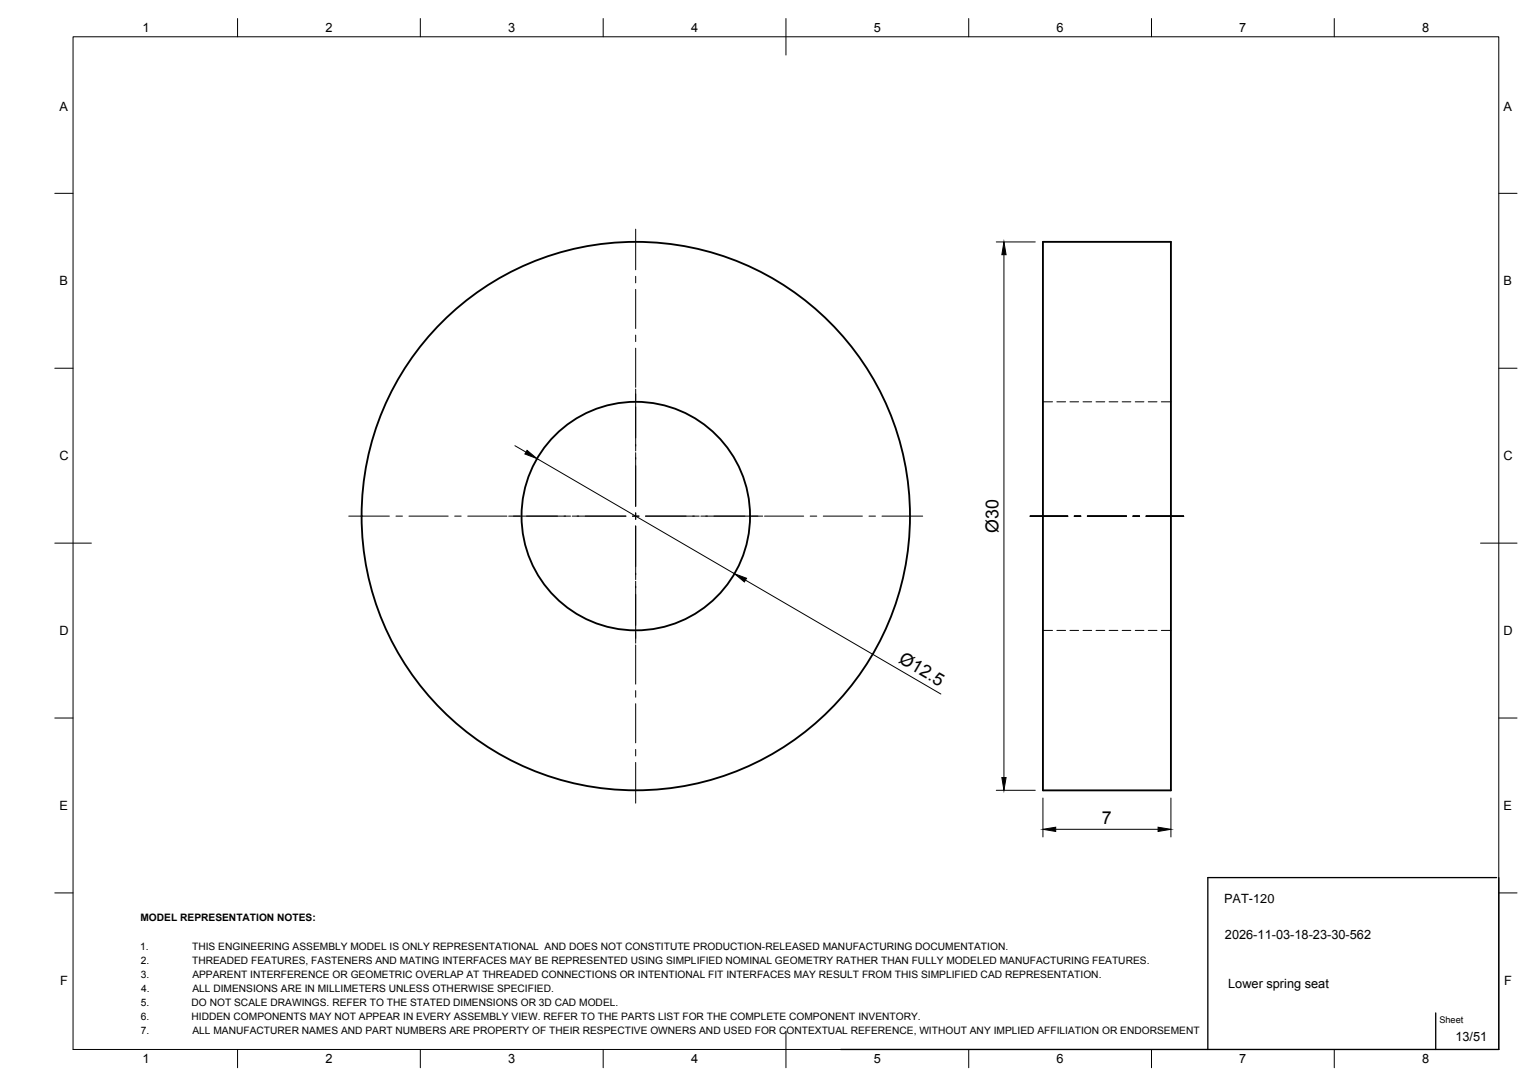
ISO-10303-21;
HEADER;
/* Generated by software containing ST-Developer
 * from STEP Tools, Inc. (www.steptools.com) 
 */

FILE_DESCRIPTION(
/* description */ ('Vibration shaker table dummy'),
/* implementation_level */ '2;1');

FILE_NAME(
/* name */ 'Lower spring seat.step',
/* time_stamp */ '2026-10-27T10:55:14-07:00',
/* author */ (''),
/* organization */ (''),
/* preprocessor_version */ 'ST-DEVELOPER v20.2',
/* originating_system */ 'Autodesk Translation Framework v15.17.0.0',
/* authorisation */ '');

FILE_SCHEMA (('AUTOMOTIVE_DESIGN { 1 0 10303 214 3 1 1 }'));
ENDSEC;

DATA;
#10=MECHANICAL_DESIGN_GEOMETRIC_PRESENTATION_REPRESENTATION('',(#694),#22394);
#602=SHAPE_REPRESENTATION_RELATIONSHIP('SRR','None',#22648,#648);
#648=ADVANCED_BREP_SHAPE_REPRESENTATION('',(#740),#22354);
#694=STYLED_ITEM('',(#22961),#740);
#740=MANIFOLD_SOLID_BREP('Body1',#9212);
#875=FACE_BOUND('',#2060,.T.);
#876=FACE_BOUND('',#2062,.T.);
#1122=PLANE('',#10011);
#1123=PLANE('',#10012);
#1459=FACE_OUTER_BOUND('',#2057,.T.);
#1460=FACE_OUTER_BOUND('',#2058,.T.);
#1461=FACE_OUTER_BOUND('',#2059,.T.);
#1462=FACE_OUTER_BOUND('',#2061,.T.);
#2057=EDGE_LOOP('',(#6810,#6811,#6812,#6813));
#2058=EDGE_LOOP('',(#6814,#6815,#6816,#6817));
#2059=EDGE_LOOP('',(#6818));
#2060=EDGE_LOOP('',(#6819));
#2061=EDGE_LOOP('',(#6820));
#2062=EDGE_LOOP('',(#6821));
#2788=LINE('',#14552,#3407);
#2789=LINE('',#14558,#3408);
#3407=VECTOR('',#11610,0.625);
#3408=VECTOR('',#11617,1.5);
#3976=CIRCLE('',#10006,0.625);
#3977=CIRCLE('',#10007,0.625);
#3978=CIRCLE('',#10009,1.5);
#3979=CIRCLE('',#10010,1.5);
#4555=VERTEX_POINT('',#14549);
#4556=VERTEX_POINT('',#14551);
#4557=VERTEX_POINT('',#14555);
#4558=VERTEX_POINT('',#14557);
#5398=EDGE_CURVE('',#4555,#4555,#3976,.T.);
#5399=EDGE_CURVE('',#4555,#4556,#2788,.T.);
#5400=EDGE_CURVE('',#4556,#4556,#3977,.T.);
#5401=EDGE_CURVE('',#4557,#4557,#3978,.T.);
#5402=EDGE_CURVE('',#4557,#4558,#2789,.T.);
#5403=EDGE_CURVE('',#4558,#4558,#3979,.T.);
#6810=ORIENTED_EDGE('',*,*,#5398,.F.);
#6811=ORIENTED_EDGE('',*,*,#5399,.T.);
#6812=ORIENTED_EDGE('',*,*,#5400,.T.);
#6813=ORIENTED_EDGE('',*,*,#5399,.F.);
#6814=ORIENTED_EDGE('',*,*,#5401,.F.);
#6815=ORIENTED_EDGE('',*,*,#5402,.T.);
#6816=ORIENTED_EDGE('',*,*,#5403,.T.);
#6817=ORIENTED_EDGE('',*,*,#5402,.F.);
#6818=ORIENTED_EDGE('',*,*,#5401,.T.);
#6819=ORIENTED_EDGE('',*,*,#5398,.T.);
#6820=ORIENTED_EDGE('',*,*,#5403,.F.);
#6821=ORIENTED_EDGE('',*,*,#5400,.F.);
#8562=CYLINDRICAL_SURFACE('',#10005,0.625);
#8563=CYLINDRICAL_SURFACE('',#10008,1.5);
#8824=ADVANCED_FACE('',(#1459),#8562,.F.);
#8825=ADVANCED_FACE('',(#1460),#8563,.T.);
#8826=ADVANCED_FACE('',(#1461,#875),#1122,.T.);
#8827=ADVANCED_FACE('',(#1462,#876),#1123,.F.);
#9212=CLOSED_SHELL('',(#8824,#8825,#8826,#8827));
#10004=AXIS2_PLACEMENT_3D('',#14547,#11604,#11605);
#10005=AXIS2_PLACEMENT_3D('',#14548,#11606,#11607);
#10006=AXIS2_PLACEMENT_3D('',#14550,#11608,#11609);
#10007=AXIS2_PLACEMENT_3D('',#14553,#11611,#11612);
#10008=AXIS2_PLACEMENT_3D('',#14554,#11613,#11614);
#10009=AXIS2_PLACEMENT_3D('',#14556,#11615,#11616);
#10010=AXIS2_PLACEMENT_3D('',#14559,#11618,#11619);
#10011=AXIS2_PLACEMENT_3D('',#14560,#11620,#11621);
#10012=AXIS2_PLACEMENT_3D('',#14561,#11622,#11623);
#11604=DIRECTION('axis',(0.,0.,1.));
#11605=DIRECTION('refdir',(1.,0.,0.));
#11606=DIRECTION('center_axis',(0.,0.,1.));
#11607=DIRECTION('ref_axis',(1.,0.,0.));
#11608=DIRECTION('center_axis',(0.,0.,-1.));
#11609=DIRECTION('ref_axis',(1.,0.,0.));
#11610=DIRECTION('',(0.,0.,-1.));
#11611=DIRECTION('center_axis',(0.,0.,-1.));
#11612=DIRECTION('ref_axis',(1.,0.,0.));
#11613=DIRECTION('center_axis',(0.,0.,1.));
#11614=DIRECTION('ref_axis',(1.,0.,0.));
#11615=DIRECTION('center_axis',(0.,0.,1.));
#11616=DIRECTION('ref_axis',(1.,0.,0.));
#11617=DIRECTION('',(0.,0.,-1.));
#11618=DIRECTION('center_axis',(0.,0.,1.));
#11619=DIRECTION('ref_axis',(1.,0.,0.));
#11620=DIRECTION('center_axis',(0.,0.,1.));
#11621=DIRECTION('ref_axis',(1.,0.,0.));
#11622=DIRECTION('center_axis',(0.,0.,1.));
#11623=DIRECTION('ref_axis',(1.,0.,0.));
#14547=CARTESIAN_POINT('',(0.,0.,0.));
#14548=CARTESIAN_POINT('Origin',(-6.,-4.,1.9));
#14549=CARTESIAN_POINT('',(-6.625,-4.,2.6));
#14550=CARTESIAN_POINT('Origin',(-6.,-4.,2.6));
#14551=CARTESIAN_POINT('',(-6.625,-4.,1.9));
#14552=CARTESIAN_POINT('',(-6.625,-4.,1.9));
#14553=CARTESIAN_POINT('Origin',(-6.,-4.,1.9));
#14554=CARTESIAN_POINT('Origin',(-6.,-4.,1.9));
#14555=CARTESIAN_POINT('',(-7.5,-4.,2.6));
#14556=CARTESIAN_POINT('Origin',(-6.,-4.,2.6));
#14557=CARTESIAN_POINT('',(-7.5,-4.,1.9));
#14558=CARTESIAN_POINT('',(-7.5,-4.,1.9));
#14559=CARTESIAN_POINT('Origin',(-6.,-4.,1.9));
#14560=CARTESIAN_POINT('Origin',(-6.,-4.,2.6));
#14561=CARTESIAN_POINT('Origin',(-6.,-4.,1.9));
#22303=UNCERTAINTY_MEASURE_WITH_UNIT(LENGTH_MEASURE(0.001),#22395,
'DISTANCE_ACCURACY_VALUE',
'Maximum model space distance between geometric entities at asserted c
onnectivities');
#22343=UNCERTAINTY_MEASURE_WITH_UNIT(LENGTH_MEASURE(0.001),#22395,
'DISTANCE_ACCURACY_VALUE',
'Maximum model space distance between geometric entities at asserted c
onnectivities');
#22354=(
GEOMETRIC_REPRESENTATION_CONTEXT(3)
GLOBAL_UNCERTAINTY_ASSIGNED_CONTEXT((#22303))
GLOBAL_UNIT_ASSIGNED_CONTEXT((#22395,#22397,#22398))
REPRESENTATION_CONTEXT('','3D')
);
#22394=(
GEOMETRIC_REPRESENTATION_CONTEXT(3)
GLOBAL_UNCERTAINTY_ASSIGNED_CONTEXT((#22343))
GLOBAL_UNIT_ASSIGNED_CONTEXT((#22395,#22397,#22398))
REPRESENTATION_CONTEXT('','3D')
);
#22395=(
LENGTH_UNIT()
NAMED_UNIT(*)
SI_UNIT(.CENTI.,.METRE.)
);
#22397=(
NAMED_UNIT(*)
PLANE_ANGLE_UNIT()
SI_UNIT($,.RADIAN.)
);
#22398=(
NAMED_UNIT(*)
SI_UNIT($,.STERADIAN.)
SOLID_ANGLE_UNIT()
);
#22409=SHAPE_DEFINITION_REPRESENTATION(#22459,#22648);
#22459=PRODUCT_DEFINITION_SHAPE('',$,#22699);
#22648=SHAPE_REPRESENTATION('',(#10004),#22354);
#22688=PRODUCT_DEFINITION_CONTEXT('part definition',#22840,'design');
#22699=PRODUCT_DEFINITION('Lower spring seat','Lower spring seat',#22749,
#22688);
#22749=PRODUCT_DEFINITION_FORMATION('',$,#22852);
#22840=APPLICATION_CONTEXT(
'Core Data for Automotive Mechanical Design Process');
#22841=PRODUCT_CONTEXT('part definition',#22840,'mechanical');
#22852=PRODUCT('Lower spring seat','Lower spring seat',
'Lower spring seat',(#22841));
#22955=COLOUR_RGB('Grey',0.48,0.52,0.57);
#22956=FILL_AREA_STYLE_COLOUR('',#22955);
#22957=FILL_AREA_STYLE('',(#22956));
#22958=SURFACE_STYLE_FILL_AREA(#22957);
#22959=SURFACE_SIDE_STYLE('',(#22958));
#22960=SURFACE_STYLE_USAGE(.BOTH.,#22959);
#22961=PRESENTATION_STYLE_ASSIGNMENT((#22960));
ENDSEC;
END-ISO-10303-21;
